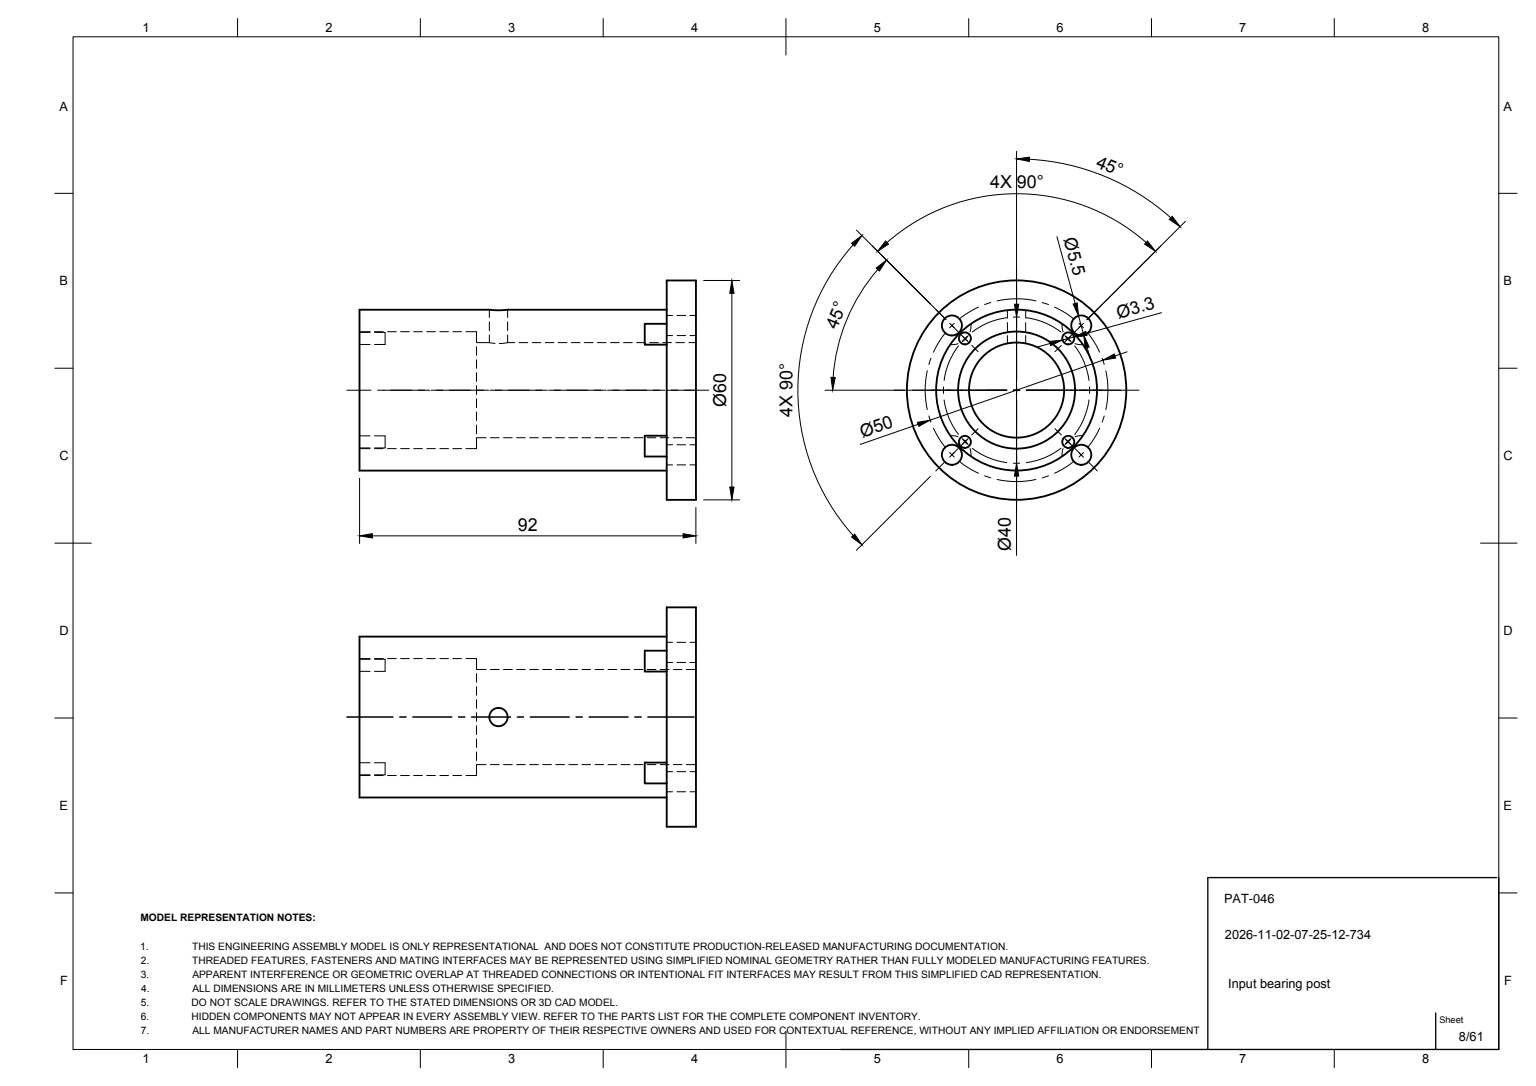
ISO-10303-21;
HEADER;
/* Generated by software containing ST-Developer
 * from STEP Tools, Inc. (www.steptools.com) 
 */

FILE_DESCRIPTION(
/* description */ ('Gear mesh backlash fixture'),
/* implementation_level */ '2;1');

FILE_NAME(
/* name */ 'Input bearing post.step',
/* time_stamp */ '2026-10-28T03:26:00-07:00',
/* author */ (''),
/* organization */ (''),
/* preprocessor_version */ 'ST-DEVELOPER v20.2',
/* originating_system */ 'Autodesk Translation Framework v15.17.0.0',
/* authorisation */ '');

FILE_SCHEMA (('AUTOMOTIVE_DESIGN { 1 0 10303 214 3 1 1 }'));
ENDSEC;

DATA;
#10=MECHANICAL_DESIGN_GEOMETRIC_PRESENTATION_REPRESENTATION('',(#1019),#57900);
#784=B_SPLINE_CURVE_WITH_KNOTS('',3,(#19392,#19393,#19394,#19395,#19396,
#19397,#19398,#19399,#19400,#19401),.UNSPECIFIED.,.F.,.F.,(4,2,2,2,4),(0.,
0.0944273339541119,0.188854667908224,0.283277491997423,0.377700316086621),
 .UNSPECIFIED.);
#785=B_SPLINE_CURVE_WITH_KNOTS('',3,(#19402,#19403,#19404,#19405,#19406,
#19407,#19408,#19409,#19410,#19411,#19412,#19413,#19414,#19415,#19416,#19417,
#19418,#19419,#19420,#19421,#19422,#19423,#19424,#19425,#19426,#19427),
 .UNSPECIFIED.,.F.,.F.,(4,2,2,2,2,2,2,2,2,2,2,2,4),(0.377700316086621,0.47212314017582,
0.56654596426502,0.660973298219131,0.755400632173242,0.849827966127354,
0.944255300081465,1.03867812417066,1.13310094825986,1.22752377234906,1.32194659643826,
1.41637393039237,1.51080126434648),.UNSPECIFIED.);
#786=B_SPLINE_CURVE_WITH_KNOTS('',3,(#19431,#19432,#19433,#19434,#19435,
#19436,#19437,#19438,#19439,#19440,#19441,#19442,#19443,#19444,#19445,#19446,
#19447,#19448,#19449,#19450,#19451,#19452,#19453,#19454,#19455,#19456),
 .UNSPECIFIED.,.F.,.F.,(4,2,2,2,2,2,2,2,2,2,2,2,4),(0.,0.0942593862034407,
0.188518772406881,0.282777622143722,0.377036471880563,0.471295321617403,
0.565554171354244,0.659813557557685,0.754072943761126,0.848332329964567,
0.942591716168009,1.03685056590485,1.13110941564169),.UNSPECIFIED.);
#787=B_SPLINE_CURVE_WITH_KNOTS('',3,(#19457,#19458,#19459,#19460,#19461,
#19462,#19463,#19464,#19465,#19466),.UNSPECIFIED.,.F.,.F.,(4,2,2,2,4),(1.13110941564169,
1.22536826537853,1.31962711511537,1.41388650131881,1.50814588752225),
 .UNSPECIFIED.);
#919=SHAPE_REPRESENTATION_RELATIONSHIP('SRR','None',#58114,#969);
#969=ADVANCED_BREP_SHAPE_REPRESENTATION('',(#1084),#57847);
#1019=STYLED_ITEM('',(#58465),#1084);
#1084=MANIFOLD_SOLID_BREP('Body1',#13579);
#1167=FACE_BOUND('',#2531,.T.);
#1168=FACE_BOUND('',#2533,.T.);
#1169=FACE_BOUND('',#2534,.T.);
#1170=FACE_BOUND('',#2535,.T.);
#1171=FACE_BOUND('',#2536,.T.);
#1172=FACE_BOUND('',#2537,.T.);
#1173=FACE_BOUND('',#2544,.T.);
#1174=FACE_BOUND('',#2547,.T.);
#1175=FACE_BOUND('',#2549,.T.);
#1176=FACE_BOUND('',#2550,.T.);
#1177=FACE_BOUND('',#2551,.T.);
#1178=FACE_BOUND('',#2552,.T.);
#1179=FACE_BOUND('',#2553,.T.);
#1180=FACE_BOUND('',#2555,.T.);
#1181=FACE_BOUND('',#2556,.T.);
#1182=FACE_BOUND('',#2557,.T.);
#1183=FACE_BOUND('',#2558,.T.);
#1184=FACE_BOUND('',#2559,.T.);
#1348=PLANE('',#14259);
#1349=PLANE('',#14263);
#1350=PLANE('',#14267);
#1351=PLANE('',#14271);
#1352=PLANE('',#14272);
#1353=PLANE('',#14280);
#1354=PLANE('',#14285);
#1355=PLANE('',#14290);
#1356=PLANE('',#14299);
#1357=PLANE('',#14316);
#1358=PLANE('',#14322);
#1359=PLANE('',#14323);
#1724=FACE_OUTER_BOUND('',#2513,.T.);
#1725=FACE_OUTER_BOUND('',#2514,.T.);
#1726=FACE_OUTER_BOUND('',#2515,.T.);
#1727=FACE_OUTER_BOUND('',#2516,.T.);
#1728=FACE_OUTER_BOUND('',#2517,.T.);
#1729=FACE_OUTER_BOUND('',#2518,.T.);
#1730=FACE_OUTER_BOUND('',#2519,.T.);
#1731=FACE_OUTER_BOUND('',#2520,.T.);
#1732=FACE_OUTER_BOUND('',#2521,.T.);
#1733=FACE_OUTER_BOUND('',#2522,.T.);
#1734=FACE_OUTER_BOUND('',#2523,.T.);
#1735=FACE_OUTER_BOUND('',#2524,.T.);
#1736=FACE_OUTER_BOUND('',#2525,.T.);
#1737=FACE_OUTER_BOUND('',#2526,.T.);
#1738=FACE_OUTER_BOUND('',#2527,.T.);
#1739=FACE_OUTER_BOUND('',#2528,.T.);
#1740=FACE_OUTER_BOUND('',#2529,.T.);
#1741=FACE_OUTER_BOUND('',#2530,.T.);
#1742=FACE_OUTER_BOUND('',#2532,.T.);
#1743=FACE_OUTER_BOUND('',#2538,.T.);
#1744=FACE_OUTER_BOUND('',#2539,.T.);
#1745=FACE_OUTER_BOUND('',#2540,.T.);
#1746=FACE_OUTER_BOUND('',#2541,.T.);
#1747=FACE_OUTER_BOUND('',#2542,.T.);
#1748=FACE_OUTER_BOUND('',#2543,.T.);
#1749=FACE_OUTER_BOUND('',#2545,.T.);
#1750=FACE_OUTER_BOUND('',#2546,.T.);
#1751=FACE_OUTER_BOUND('',#2548,.T.);
#1752=FACE_OUTER_BOUND('',#2554,.T.);
#2513=EDGE_LOOP('',(#9023,#9024,#9025,#9026,#9027,#9028));
#2514=EDGE_LOOP('',(#9029,#9030,#9031,#9032));
#2515=EDGE_LOOP('',(#9033));
#2516=EDGE_LOOP('',(#9034,#9035,#9036,#9037));
#2517=EDGE_LOOP('',(#9038));
#2518=EDGE_LOOP('',(#9039,#9040,#9041,#9042));
#2519=EDGE_LOOP('',(#9043));
#2520=EDGE_LOOP('',(#9044,#9045,#9046,#9047));
#2521=EDGE_LOOP('',(#9048));
#2522=EDGE_LOOP('',(#9049,#9050));
#2523=EDGE_LOOP('',(#9051,#9052,#9053,#9054));
#2524=EDGE_LOOP('',(#9055,#9056,#9057,#9058));
#2525=EDGE_LOOP('',(#9059,#9060));
#2526=EDGE_LOOP('',(#9061,#9062,#9063,#9064));
#2527=EDGE_LOOP('',(#9065,#9066));
#2528=EDGE_LOOP('',(#9067,#9068,#9069,#9070));
#2529=EDGE_LOOP('',(#9071,#9072));
#2530=EDGE_LOOP('',(#9073,#9074,#9075,#9076,#9077,#9078,#9079,#9080,#9081,
#9082,#9083,#9084,#9085,#9086,#9087,#9088,#9089,#9090,#9091,#9092));
#2531=EDGE_LOOP('',(#9093,#9094));
#2532=EDGE_LOOP('',(#9095));
#2533=EDGE_LOOP('',(#9096,#9097,#9098,#9099,#9100,#9101,#9102,#9103,#9104));
#2534=EDGE_LOOP('',(#9105));
#2535=EDGE_LOOP('',(#9106));
#2536=EDGE_LOOP('',(#9107));
#2537=EDGE_LOOP('',(#9108));
#2538=EDGE_LOOP('',(#9109,#9110,#9111,#9112));
#2539=EDGE_LOOP('',(#9113,#9114,#9115,#9116));
#2540=EDGE_LOOP('',(#9117,#9118,#9119,#9120));
#2541=EDGE_LOOP('',(#9121,#9122,#9123,#9124));
#2542=EDGE_LOOP('',(#9125,#9126,#9127,#9128));
#2543=EDGE_LOOP('',(#9129));
#2544=EDGE_LOOP('',(#9130));
#2545=EDGE_LOOP('',(#9131,#9132,#9133,#9134));
#2546=EDGE_LOOP('',(#9135,#9136,#9137,#9138));
#2547=EDGE_LOOP('',(#9139,#9140));
#2548=EDGE_LOOP('',(#9141));
#2549=EDGE_LOOP('',(#9142));
#2550=EDGE_LOOP('',(#9143));
#2551=EDGE_LOOP('',(#9144));
#2552=EDGE_LOOP('',(#9145));
#2553=EDGE_LOOP('',(#9146));
#2554=EDGE_LOOP('',(#9147));
#2555=EDGE_LOOP('',(#9148));
#2556=EDGE_LOOP('',(#9149));
#2557=EDGE_LOOP('',(#9150));
#2558=EDGE_LOOP('',(#9151));
#2559=EDGE_LOOP('',(#9152));
#3459=LINE('',#19429,#4348);
#3460=LINE('',#19471,#4349);
#3461=LINE('',#19478,#4350);
#3462=LINE('',#19485,#4351);
#3463=LINE('',#19492,#4352);
#3464=LINE('',#19502,#4353);
#3465=LINE('',#19505,#4354);
#3466=LINE('',#19509,#4355);
#3467=LINE('',#19513,#4356);
#3468=LINE('',#19520,#4357);
#3469=LINE('',#19524,#4358);
#3470=LINE('',#19531,#4359);
#3471=LINE('',#19535,#4360);
#3472=LINE('',#19543,#4361);
#3473=LINE('',#19563,#4362);
#3474=LINE('',#19567,#4363);
#3475=LINE('',#19571,#4364);
#3476=LINE('',#19575,#4365);
#3477=LINE('',#19580,#4366);
#3478=LINE('',#19587,#4367);
#3479=LINE('',#19591,#4368);
#4348=VECTOR('',#15748,0.25);
#4349=VECTOR('',#15753,0.165);
#4350=VECTOR('',#15762,0.165);
#4351=VECTOR('',#15771,0.165);
#4352=VECTOR('',#15780,0.165);
#4353=VECTOR('',#15793,1.);
#4354=VECTOR('',#15796,1.);
#4355=VECTOR('',#15799,1.);
#4356=VECTOR('',#15802,1.);
#4357=VECTOR('',#15811,1.);
#4358=VECTOR('',#15814,1.);
#4359=VECTOR('',#15823,1.);
#4360=VECTOR('',#15826,1.);
#4361=VECTOR('',#15837,2.2);
#4362=VECTOR('',#15864,0.275);
#4363=VECTOR('',#15869,0.275);
#4364=VECTOR('',#15874,0.275);
#4365=VECTOR('',#15879,0.275);
#4366=VECTOR('',#15884,1.6);
#4367=VECTOR('',#15893,3.);
#4368=VECTOR('',#15898,1.3);
#5213=CIRCLE('',#14257,0.165);
#5214=CIRCLE('',#14258,0.165);
#5215=CIRCLE('',#14261,0.165);
#5216=CIRCLE('',#14262,0.165);
#5217=CIRCLE('',#14265,0.165);
#5218=CIRCLE('',#14266,0.165);
#5219=CIRCLE('',#14269,0.165);
#5220=CIRCLE('',#14270,0.165);
#5221=CIRCLE('',#14273,2.2);
#5222=CIRCLE('',#14274,0.525);
#5223=CIRCLE('',#14276,0.525);
#5224=CIRCLE('',#14278,0.525);
#5225=CIRCLE('',#14279,0.525);
#5226=CIRCLE('',#14281,2.2);
#5227=CIRCLE('',#14283,0.525);
#5228=CIRCLE('',#14284,0.525);
#5229=CIRCLE('',#14286,2.2);
#5230=CIRCLE('',#14288,0.525);
#5231=CIRCLE('',#14289,0.525);
#5232=CIRCLE('',#14291,2.2);
#5233=CIRCLE('',#14293,2.2);
#5234=CIRCLE('',#14294,2.2);
#5235=CIRCLE('',#14295,2.2);
#5236=CIRCLE('',#14296,2.2);
#5237=CIRCLE('',#14297,2.2);
#5238=CIRCLE('',#14298,2.2);
#5239=CIRCLE('',#14300,3.);
#5240=CIRCLE('',#14301,0.275);
#5241=CIRCLE('',#14302,0.275);
#5242=CIRCLE('',#14303,0.275);
#5243=CIRCLE('',#14304,0.275);
#5244=CIRCLE('',#14306,0.275);
#5245=CIRCLE('',#14308,0.275);
#5246=CIRCLE('',#14310,0.275);
#5247=CIRCLE('',#14312,0.275);
#5248=CIRCLE('',#14314,1.6);
#5249=CIRCLE('',#14315,1.6);
#5250=CIRCLE('',#14317,1.3);
#5251=CIRCLE('',#14319,3.);
#5252=CIRCLE('',#14321,1.3);
#5829=VERTEX_POINT('',#19390);
#5830=VERTEX_POINT('',#19391);
#5831=VERTEX_POINT('',#19428);
#5832=VERTEX_POINT('',#19430);
#5833=VERTEX_POINT('',#19468);
#5834=VERTEX_POINT('',#19470);
#5835=VERTEX_POINT('',#19475);
#5836=VERTEX_POINT('',#19477);
#5837=VERTEX_POINT('',#19482);
#5838=VERTEX_POINT('',#19484);
#5839=VERTEX_POINT('',#19489);
#5840=VERTEX_POINT('',#19491);
#5841=VERTEX_POINT('',#19496);
#5842=VERTEX_POINT('',#19497);
#5843=VERTEX_POINT('',#19501);
#5844=VERTEX_POINT('',#19503);
#5845=VERTEX_POINT('',#19507);
#5846=VERTEX_POINT('',#19508);
#5847=VERTEX_POINT('',#19510);
#5848=VERTEX_POINT('',#19512);
#5849=VERTEX_POINT('',#19518);
#5850=VERTEX_POINT('',#19519);
#5851=VERTEX_POINT('',#19521);
#5852=VERTEX_POINT('',#19523);
#5853=VERTEX_POINT('',#19529);
#5854=VERTEX_POINT('',#19530);
#5855=VERTEX_POINT('',#19532);
#5856=VERTEX_POINT('',#19534);
#5857=VERTEX_POINT('',#19540);
#5858=VERTEX_POINT('',#19542);
#5859=VERTEX_POINT('',#19550);
#5860=VERTEX_POINT('',#19552);
#5861=VERTEX_POINT('',#19554);
#5862=VERTEX_POINT('',#19556);
#5863=VERTEX_POINT('',#19558);
#5864=VERTEX_POINT('',#19561);
#5865=VERTEX_POINT('',#19565);
#5866=VERTEX_POINT('',#19569);
#5867=VERTEX_POINT('',#19573);
#5868=VERTEX_POINT('',#19577);
#5869=VERTEX_POINT('',#19579);
#5870=VERTEX_POINT('',#19583);
#5871=VERTEX_POINT('',#19586);
#5872=VERTEX_POINT('',#19590);
#7098=EDGE_CURVE('',#5829,#5830,#784,.T.);
#7099=EDGE_CURVE('',#5830,#5829,#785,.T.);
#7100=EDGE_CURVE('',#5830,#5831,#3459,.T.);
#7101=EDGE_CURVE('',#5832,#5831,#786,.T.);
#7102=EDGE_CURVE('',#5831,#5832,#787,.T.);
#7103=EDGE_CURVE('',#5833,#5833,#5213,.T.);
#7104=EDGE_CURVE('',#5833,#5834,#3460,.T.);
#7105=EDGE_CURVE('',#5834,#5834,#5214,.T.);
#7106=EDGE_CURVE('',#5835,#5835,#5215,.T.);
#7107=EDGE_CURVE('',#5835,#5836,#3461,.T.);
#7108=EDGE_CURVE('',#5836,#5836,#5216,.T.);
#7109=EDGE_CURVE('',#5837,#5837,#5217,.T.);
#7110=EDGE_CURVE('',#5837,#5838,#3462,.T.);
#7111=EDGE_CURVE('',#5838,#5838,#5218,.T.);
#7112=EDGE_CURVE('',#5839,#5839,#5219,.T.);
#7113=EDGE_CURVE('',#5839,#5840,#3463,.T.);
#7114=EDGE_CURVE('',#5840,#5840,#5220,.T.);
#7115=EDGE_CURVE('',#5841,#5842,#5221,.T.);
#7116=EDGE_CURVE('',#5842,#5841,#5222,.T.);
#7117=EDGE_CURVE('',#5843,#5841,#3464,.T.);
#7118=EDGE_CURVE('',#5844,#5843,#5223,.T.);
#7119=EDGE_CURVE('',#5842,#5844,#3465,.T.);
#7120=EDGE_CURVE('',#5845,#5846,#3466,.T.);
#7121=EDGE_CURVE('',#5845,#5847,#5224,.T.);
#7122=EDGE_CURVE('',#5848,#5847,#3467,.T.);
#7123=EDGE_CURVE('',#5846,#5848,#5225,.T.);
#7124=EDGE_CURVE('',#5847,#5845,#5226,.T.);
#7125=EDGE_CURVE('',#5849,#5850,#3468,.T.);
#7126=EDGE_CURVE('',#5849,#5851,#5227,.T.);
#7127=EDGE_CURVE('',#5852,#5851,#3469,.T.);
#7128=EDGE_CURVE('',#5850,#5852,#5228,.T.);
#7129=EDGE_CURVE('',#5851,#5849,#5229,.T.);
#7130=EDGE_CURVE('',#5853,#5854,#3470,.T.);
#7131=EDGE_CURVE('',#5853,#5855,#5230,.T.);
#7132=EDGE_CURVE('',#5856,#5855,#3471,.T.);
#7133=EDGE_CURVE('',#5854,#5856,#5231,.T.);
#7134=EDGE_CURVE('',#5855,#5853,#5232,.T.);
#7135=EDGE_CURVE('',#5857,#5857,#5233,.T.);
#7136=EDGE_CURVE('',#5857,#5858,#3472,.T.);
#7137=EDGE_CURVE('',#5858,#5843,#5234,.T.);
#7138=EDGE_CURVE('',#5844,#5856,#5235,.T.);
#7139=EDGE_CURVE('',#5854,#5852,#5236,.T.);
#7140=EDGE_CURVE('',#5850,#5848,#5237,.T.);
#7141=EDGE_CURVE('',#5846,#5858,#5238,.T.);
#7142=EDGE_CURVE('',#5859,#5859,#5239,.T.);
#7143=EDGE_CURVE('',#5860,#5860,#5240,.T.);
#7144=EDGE_CURVE('',#5861,#5861,#5241,.T.);
#7145=EDGE_CURVE('',#5862,#5862,#5242,.T.);
#7146=EDGE_CURVE('',#5863,#5863,#5243,.T.);
#7147=EDGE_CURVE('',#5864,#5864,#5244,.T.);
#7148=EDGE_CURVE('',#5864,#5860,#3473,.T.);
#7149=EDGE_CURVE('',#5865,#5865,#5245,.T.);
#7150=EDGE_CURVE('',#5865,#5863,#3474,.T.);
#7151=EDGE_CURVE('',#5866,#5866,#5246,.T.);
#7152=EDGE_CURVE('',#5866,#5861,#3475,.T.);
#7153=EDGE_CURVE('',#5867,#5867,#5247,.T.);
#7154=EDGE_CURVE('',#5867,#5862,#3476,.T.);
#7155=EDGE_CURVE('',#5868,#5868,#5248,.T.);
#7156=EDGE_CURVE('',#5868,#5869,#3477,.T.);
#7157=EDGE_CURVE('',#5869,#5869,#5249,.T.);
#7158=EDGE_CURVE('',#5870,#5870,#5250,.T.);
#7159=EDGE_CURVE('',#5859,#5871,#3478,.T.);
#7160=EDGE_CURVE('',#5871,#5871,#5251,.T.);
#7161=EDGE_CURVE('',#5870,#5872,#3479,.T.);
#7162=EDGE_CURVE('',#5872,#5872,#5252,.T.);
#9023=ORIENTED_EDGE('',*,*,#7098,.F.);
#9024=ORIENTED_EDGE('',*,*,#7099,.F.);
#9025=ORIENTED_EDGE('',*,*,#7100,.T.);
#9026=ORIENTED_EDGE('',*,*,#7101,.F.);
#9027=ORIENTED_EDGE('',*,*,#7102,.F.);
#9028=ORIENTED_EDGE('',*,*,#7100,.F.);
#9029=ORIENTED_EDGE('',*,*,#7103,.F.);
#9030=ORIENTED_EDGE('',*,*,#7104,.T.);
#9031=ORIENTED_EDGE('',*,*,#7105,.F.);
#9032=ORIENTED_EDGE('',*,*,#7104,.F.);
#9033=ORIENTED_EDGE('',*,*,#7103,.T.);
#9034=ORIENTED_EDGE('',*,*,#7106,.F.);
#9035=ORIENTED_EDGE('',*,*,#7107,.T.);
#9036=ORIENTED_EDGE('',*,*,#7108,.F.);
#9037=ORIENTED_EDGE('',*,*,#7107,.F.);
#9038=ORIENTED_EDGE('',*,*,#7106,.T.);
#9039=ORIENTED_EDGE('',*,*,#7109,.F.);
#9040=ORIENTED_EDGE('',*,*,#7110,.T.);
#9041=ORIENTED_EDGE('',*,*,#7111,.F.);
#9042=ORIENTED_EDGE('',*,*,#7110,.F.);
#9043=ORIENTED_EDGE('',*,*,#7109,.T.);
#9044=ORIENTED_EDGE('',*,*,#7112,.F.);
#9045=ORIENTED_EDGE('',*,*,#7113,.T.);
#9046=ORIENTED_EDGE('',*,*,#7114,.F.);
#9047=ORIENTED_EDGE('',*,*,#7113,.F.);
#9048=ORIENTED_EDGE('',*,*,#7112,.T.);
#9049=ORIENTED_EDGE('',*,*,#7115,.F.);
#9050=ORIENTED_EDGE('',*,*,#7116,.F.);
#9051=ORIENTED_EDGE('',*,*,#7117,.F.);
#9052=ORIENTED_EDGE('',*,*,#7118,.F.);
#9053=ORIENTED_EDGE('',*,*,#7119,.F.);
#9054=ORIENTED_EDGE('',*,*,#7116,.T.);
#9055=ORIENTED_EDGE('',*,*,#7120,.F.);
#9056=ORIENTED_EDGE('',*,*,#7121,.T.);
#9057=ORIENTED_EDGE('',*,*,#7122,.F.);
#9058=ORIENTED_EDGE('',*,*,#7123,.F.);
#9059=ORIENTED_EDGE('',*,*,#7124,.F.);
#9060=ORIENTED_EDGE('',*,*,#7121,.F.);
#9061=ORIENTED_EDGE('',*,*,#7125,.F.);
#9062=ORIENTED_EDGE('',*,*,#7126,.T.);
#9063=ORIENTED_EDGE('',*,*,#7127,.F.);
#9064=ORIENTED_EDGE('',*,*,#7128,.F.);
#9065=ORIENTED_EDGE('',*,*,#7129,.F.);
#9066=ORIENTED_EDGE('',*,*,#7126,.F.);
#9067=ORIENTED_EDGE('',*,*,#7130,.F.);
#9068=ORIENTED_EDGE('',*,*,#7131,.T.);
#9069=ORIENTED_EDGE('',*,*,#7132,.F.);
#9070=ORIENTED_EDGE('',*,*,#7133,.F.);
#9071=ORIENTED_EDGE('',*,*,#7134,.F.);
#9072=ORIENTED_EDGE('',*,*,#7131,.F.);
#9073=ORIENTED_EDGE('',*,*,#7135,.F.);
#9074=ORIENTED_EDGE('',*,*,#7136,.T.);
#9075=ORIENTED_EDGE('',*,*,#7137,.T.);
#9076=ORIENTED_EDGE('',*,*,#7117,.T.);
#9077=ORIENTED_EDGE('',*,*,#7115,.T.);
#9078=ORIENTED_EDGE('',*,*,#7119,.T.);
#9079=ORIENTED_EDGE('',*,*,#7138,.T.);
#9080=ORIENTED_EDGE('',*,*,#7132,.T.);
#9081=ORIENTED_EDGE('',*,*,#7134,.T.);
#9082=ORIENTED_EDGE('',*,*,#7130,.T.);
#9083=ORIENTED_EDGE('',*,*,#7139,.T.);
#9084=ORIENTED_EDGE('',*,*,#7127,.T.);
#9085=ORIENTED_EDGE('',*,*,#7129,.T.);
#9086=ORIENTED_EDGE('',*,*,#7125,.T.);
#9087=ORIENTED_EDGE('',*,*,#7140,.T.);
#9088=ORIENTED_EDGE('',*,*,#7122,.T.);
#9089=ORIENTED_EDGE('',*,*,#7124,.T.);
#9090=ORIENTED_EDGE('',*,*,#7120,.T.);
#9091=ORIENTED_EDGE('',*,*,#7141,.T.);
#9092=ORIENTED_EDGE('',*,*,#7136,.F.);
#9093=ORIENTED_EDGE('',*,*,#7101,.T.);
#9094=ORIENTED_EDGE('',*,*,#7102,.T.);
#9095=ORIENTED_EDGE('',*,*,#7142,.T.);
#9096=ORIENTED_EDGE('',*,*,#7141,.F.);
#9097=ORIENTED_EDGE('',*,*,#7123,.T.);
#9098=ORIENTED_EDGE('',*,*,#7140,.F.);
#9099=ORIENTED_EDGE('',*,*,#7128,.T.);
#9100=ORIENTED_EDGE('',*,*,#7139,.F.);
#9101=ORIENTED_EDGE('',*,*,#7133,.T.);
#9102=ORIENTED_EDGE('',*,*,#7138,.F.);
#9103=ORIENTED_EDGE('',*,*,#7118,.T.);
#9104=ORIENTED_EDGE('',*,*,#7137,.F.);
#9105=ORIENTED_EDGE('',*,*,#7143,.T.);
#9106=ORIENTED_EDGE('',*,*,#7144,.T.);
#9107=ORIENTED_EDGE('',*,*,#7145,.T.);
#9108=ORIENTED_EDGE('',*,*,#7146,.T.);
#9109=ORIENTED_EDGE('',*,*,#7147,.F.);
#9110=ORIENTED_EDGE('',*,*,#7148,.T.);
#9111=ORIENTED_EDGE('',*,*,#7143,.F.);
#9112=ORIENTED_EDGE('',*,*,#7148,.F.);
#9113=ORIENTED_EDGE('',*,*,#7149,.F.);
#9114=ORIENTED_EDGE('',*,*,#7150,.T.);
#9115=ORIENTED_EDGE('',*,*,#7146,.F.);
#9116=ORIENTED_EDGE('',*,*,#7150,.F.);
#9117=ORIENTED_EDGE('',*,*,#7151,.F.);
#9118=ORIENTED_EDGE('',*,*,#7152,.T.);
#9119=ORIENTED_EDGE('',*,*,#7144,.F.);
#9120=ORIENTED_EDGE('',*,*,#7152,.F.);
#9121=ORIENTED_EDGE('',*,*,#7153,.F.);
#9122=ORIENTED_EDGE('',*,*,#7154,.T.);
#9123=ORIENTED_EDGE('',*,*,#7145,.F.);
#9124=ORIENTED_EDGE('',*,*,#7154,.F.);
#9125=ORIENTED_EDGE('',*,*,#7155,.F.);
#9126=ORIENTED_EDGE('',*,*,#7156,.T.);
#9127=ORIENTED_EDGE('',*,*,#7157,.F.);
#9128=ORIENTED_EDGE('',*,*,#7156,.F.);
#9129=ORIENTED_EDGE('',*,*,#7155,.T.);
#9130=ORIENTED_EDGE('',*,*,#7158,.F.);
#9131=ORIENTED_EDGE('',*,*,#7142,.F.);
#9132=ORIENTED_EDGE('',*,*,#7159,.T.);
#9133=ORIENTED_EDGE('',*,*,#7160,.T.);
#9134=ORIENTED_EDGE('',*,*,#7159,.F.);
#9135=ORIENTED_EDGE('',*,*,#7158,.T.);
#9136=ORIENTED_EDGE('',*,*,#7161,.T.);
#9137=ORIENTED_EDGE('',*,*,#7162,.T.);
#9138=ORIENTED_EDGE('',*,*,#7161,.F.);
#9139=ORIENTED_EDGE('',*,*,#7098,.T.);
#9140=ORIENTED_EDGE('',*,*,#7099,.T.);
#9141=ORIENTED_EDGE('',*,*,#7135,.T.);
#9142=ORIENTED_EDGE('',*,*,#7157,.T.);
#9143=ORIENTED_EDGE('',*,*,#7114,.T.);
#9144=ORIENTED_EDGE('',*,*,#7111,.T.);
#9145=ORIENTED_EDGE('',*,*,#7108,.T.);
#9146=ORIENTED_EDGE('',*,*,#7105,.T.);
#9147=ORIENTED_EDGE('',*,*,#7160,.F.);
#9148=ORIENTED_EDGE('',*,*,#7162,.F.);
#9149=ORIENTED_EDGE('',*,*,#7153,.T.);
#9150=ORIENTED_EDGE('',*,*,#7151,.T.);
#9151=ORIENTED_EDGE('',*,*,#7149,.T.);
#9152=ORIENTED_EDGE('',*,*,#7147,.T.);
#12597=CYLINDRICAL_SURFACE('',#14255,0.25);
#12598=CYLINDRICAL_SURFACE('',#14256,0.165);
#12599=CYLINDRICAL_SURFACE('',#14260,0.165);
#12600=CYLINDRICAL_SURFACE('',#14264,0.165);
#12601=CYLINDRICAL_SURFACE('',#14268,0.165);
#12602=CYLINDRICAL_SURFACE('',#14275,0.525);
#12603=CYLINDRICAL_SURFACE('',#14277,0.525);
#12604=CYLINDRICAL_SURFACE('',#14282,0.525);
#12605=CYLINDRICAL_SURFACE('',#14287,0.525);
#12606=CYLINDRICAL_SURFACE('',#14292,2.2);
#12607=CYLINDRICAL_SURFACE('',#14305,0.275);
#12608=CYLINDRICAL_SURFACE('',#14307,0.275);
#12609=CYLINDRICAL_SURFACE('',#14309,0.275);
#12610=CYLINDRICAL_SURFACE('',#14311,0.275);
#12611=CYLINDRICAL_SURFACE('',#14313,1.6);
#12612=CYLINDRICAL_SURFACE('',#14318,3.);
#12613=CYLINDRICAL_SURFACE('',#14320,1.3);
#12841=ADVANCED_FACE('',(#1724),#12597,.F.);
#12842=ADVANCED_FACE('',(#1725),#12598,.F.);
#12843=ADVANCED_FACE('',(#1726),#1348,.T.);
#12844=ADVANCED_FACE('',(#1727),#12599,.F.);
#12845=ADVANCED_FACE('',(#1728),#1349,.T.);
#12846=ADVANCED_FACE('',(#1729),#12600,.F.);
#12847=ADVANCED_FACE('',(#1730),#1350,.T.);
#12848=ADVANCED_FACE('',(#1731),#12601,.F.);
#12849=ADVANCED_FACE('',(#1732),#1351,.T.);
#12850=ADVANCED_FACE('',(#1733),#1352,.F.);
#12851=ADVANCED_FACE('',(#1734),#12602,.F.);
#12852=ADVANCED_FACE('',(#1735),#12603,.F.);
#12853=ADVANCED_FACE('',(#1736),#1353,.F.);
#12854=ADVANCED_FACE('',(#1737),#12604,.F.);
#12855=ADVANCED_FACE('',(#1738),#1354,.F.);
#12856=ADVANCED_FACE('',(#1739),#12605,.F.);
#12857=ADVANCED_FACE('',(#1740),#1355,.F.);
#12858=ADVANCED_FACE('',(#1741,#1167),#12606,.T.);
#12859=ADVANCED_FACE('',(#1742,#1168,#1169,#1170,#1171,#1172),#1356,.T.);
#12860=ADVANCED_FACE('',(#1743),#12607,.F.);
#12861=ADVANCED_FACE('',(#1744),#12608,.F.);
#12862=ADVANCED_FACE('',(#1745),#12609,.F.);
#12863=ADVANCED_FACE('',(#1746),#12610,.F.);
#12864=ADVANCED_FACE('',(#1747),#12611,.F.);
#12865=ADVANCED_FACE('',(#1748,#1173),#1357,.T.);
#12866=ADVANCED_FACE('',(#1749),#12612,.T.);
#12867=ADVANCED_FACE('',(#1750,#1174),#12613,.F.);
#12868=ADVANCED_FACE('',(#1751,#1175,#1176,#1177,#1178,#1179),#1358,.T.);
#12869=ADVANCED_FACE('',(#1752,#1180,#1181,#1182,#1183,#1184),#1359,.F.);
#13579=CLOSED_SHELL('',(#12841,#12842,#12843,#12844,#12845,#12846,#12847,
#12848,#12849,#12850,#12851,#12852,#12853,#12854,#12855,#12856,#12857,#12858,
#12859,#12860,#12861,#12862,#12863,#12864,#12865,#12866,#12867,#12868,#12869));
#14254=AXIS2_PLACEMENT_3D('',#19388,#15744,#15745);
#14255=AXIS2_PLACEMENT_3D('',#19389,#15746,#15747);
#14256=AXIS2_PLACEMENT_3D('',#19467,#15749,#15750);
#14257=AXIS2_PLACEMENT_3D('',#19469,#15751,#15752);
#14258=AXIS2_PLACEMENT_3D('',#19472,#15754,#15755);
#14259=AXIS2_PLACEMENT_3D('',#19473,#15756,#15757);
#14260=AXIS2_PLACEMENT_3D('',#19474,#15758,#15759);
#14261=AXIS2_PLACEMENT_3D('',#19476,#15760,#15761);
#14262=AXIS2_PLACEMENT_3D('',#19479,#15763,#15764);
#14263=AXIS2_PLACEMENT_3D('',#19480,#15765,#15766);
#14264=AXIS2_PLACEMENT_3D('',#19481,#15767,#15768);
#14265=AXIS2_PLACEMENT_3D('',#19483,#15769,#15770);
#14266=AXIS2_PLACEMENT_3D('',#19486,#15772,#15773);
#14267=AXIS2_PLACEMENT_3D('',#19487,#15774,#15775);
#14268=AXIS2_PLACEMENT_3D('',#19488,#15776,#15777);
#14269=AXIS2_PLACEMENT_3D('',#19490,#15778,#15779);
#14270=AXIS2_PLACEMENT_3D('',#19493,#15781,#15782);
#14271=AXIS2_PLACEMENT_3D('',#19494,#15783,#15784);
#14272=AXIS2_PLACEMENT_3D('',#19495,#15785,#15786);
#14273=AXIS2_PLACEMENT_3D('',#19498,#15787,#15788);
#14274=AXIS2_PLACEMENT_3D('',#19499,#15789,#15790);
#14275=AXIS2_PLACEMENT_3D('',#19500,#15791,#15792);
#14276=AXIS2_PLACEMENT_3D('',#19504,#15794,#15795);
#14277=AXIS2_PLACEMENT_3D('',#19506,#15797,#15798);
#14278=AXIS2_PLACEMENT_3D('',#19511,#15800,#15801);
#14279=AXIS2_PLACEMENT_3D('',#19514,#15803,#15804);
#14280=AXIS2_PLACEMENT_3D('',#19515,#15805,#15806);
#14281=AXIS2_PLACEMENT_3D('',#19516,#15807,#15808);
#14282=AXIS2_PLACEMENT_3D('',#19517,#15809,#15810);
#14283=AXIS2_PLACEMENT_3D('',#19522,#15812,#15813);
#14284=AXIS2_PLACEMENT_3D('',#19525,#15815,#15816);
#14285=AXIS2_PLACEMENT_3D('',#19526,#15817,#15818);
#14286=AXIS2_PLACEMENT_3D('',#19527,#15819,#15820);
#14287=AXIS2_PLACEMENT_3D('',#19528,#15821,#15822);
#14288=AXIS2_PLACEMENT_3D('',#19533,#15824,#15825);
#14289=AXIS2_PLACEMENT_3D('',#19536,#15827,#15828);
#14290=AXIS2_PLACEMENT_3D('',#19537,#15829,#15830);
#14291=AXIS2_PLACEMENT_3D('',#19538,#15831,#15832);
#14292=AXIS2_PLACEMENT_3D('',#19539,#15833,#15834);
#14293=AXIS2_PLACEMENT_3D('',#19541,#15835,#15836);
#14294=AXIS2_PLACEMENT_3D('',#19544,#15838,#15839);
#14295=AXIS2_PLACEMENT_3D('',#19545,#15840,#15841);
#14296=AXIS2_PLACEMENT_3D('',#19546,#15842,#15843);
#14297=AXIS2_PLACEMENT_3D('',#19547,#15844,#15845);
#14298=AXIS2_PLACEMENT_3D('',#19548,#15846,#15847);
#14299=AXIS2_PLACEMENT_3D('',#19549,#15848,#15849);
#14300=AXIS2_PLACEMENT_3D('',#19551,#15850,#15851);
#14301=AXIS2_PLACEMENT_3D('',#19553,#15852,#15853);
#14302=AXIS2_PLACEMENT_3D('',#19555,#15854,#15855);
#14303=AXIS2_PLACEMENT_3D('',#19557,#15856,#15857);
#14304=AXIS2_PLACEMENT_3D('',#19559,#15858,#15859);
#14305=AXIS2_PLACEMENT_3D('',#19560,#15860,#15861);
#14306=AXIS2_PLACEMENT_3D('',#19562,#15862,#15863);
#14307=AXIS2_PLACEMENT_3D('',#19564,#15865,#15866);
#14308=AXIS2_PLACEMENT_3D('',#19566,#15867,#15868);
#14309=AXIS2_PLACEMENT_3D('',#19568,#15870,#15871);
#14310=AXIS2_PLACEMENT_3D('',#19570,#15872,#15873);
#14311=AXIS2_PLACEMENT_3D('',#19572,#15875,#15876);
#14312=AXIS2_PLACEMENT_3D('',#19574,#15877,#15878);
#14313=AXIS2_PLACEMENT_3D('',#19576,#15880,#15881);
#14314=AXIS2_PLACEMENT_3D('',#19578,#15882,#15883);
#14315=AXIS2_PLACEMENT_3D('',#19581,#15885,#15886);
#14316=AXIS2_PLACEMENT_3D('',#19582,#15887,#15888);
#14317=AXIS2_PLACEMENT_3D('',#19584,#15889,#15890);
#14318=AXIS2_PLACEMENT_3D('',#19585,#15891,#15892);
#14319=AXIS2_PLACEMENT_3D('',#19588,#15894,#15895);
#14320=AXIS2_PLACEMENT_3D('',#19589,#15896,#15897);
#14321=AXIS2_PLACEMENT_3D('',#19592,#15899,#15900);
#14322=AXIS2_PLACEMENT_3D('',#19593,#15901,#15902);
#14323=AXIS2_PLACEMENT_3D('',#19594,#15903,#15904);
#15744=DIRECTION('axis',(0.,0.,1.));
#15745=DIRECTION('refdir',(1.,0.,0.));
#15746=DIRECTION('center_axis',(1.,0.,0.));
#15747=DIRECTION('ref_axis',(0.,0.,-1.));
#15748=DIRECTION('',(1.,0.,0.));
#15749=DIRECTION('center_axis',(0.,0.,1.));
#15750=DIRECTION('ref_axis',(1.,0.,0.));
#15751=DIRECTION('center_axis',(0.,0.,1.));
#15752=DIRECTION('ref_axis',(1.,0.,0.));
#15753=DIRECTION('',(0.,0.,1.));
#15754=DIRECTION('center_axis',(0.,0.,-1.));
#15755=DIRECTION('ref_axis',(1.,0.,0.));
#15756=DIRECTION('center_axis',(0.,0.,1.));
#15757=DIRECTION('ref_axis',(1.,0.,0.));
#15758=DIRECTION('center_axis',(0.,0.,1.));
#15759=DIRECTION('ref_axis',(1.,0.,0.));
#15760=DIRECTION('center_axis',(0.,0.,1.));
#15761=DIRECTION('ref_axis',(1.,0.,0.));
#15762=DIRECTION('',(0.,0.,1.));
#15763=DIRECTION('center_axis',(0.,0.,-1.));
#15764=DIRECTION('ref_axis',(1.,0.,0.));
#15765=DIRECTION('center_axis',(0.,0.,1.));
#15766=DIRECTION('ref_axis',(1.,0.,0.));
#15767=DIRECTION('center_axis',(0.,0.,1.));
#15768=DIRECTION('ref_axis',(1.,0.,0.));
#15769=DIRECTION('center_axis',(0.,0.,1.));
#15770=DIRECTION('ref_axis',(1.,0.,0.));
#15771=DIRECTION('',(0.,0.,1.));
#15772=DIRECTION('center_axis',(0.,0.,-1.));
#15773=DIRECTION('ref_axis',(1.,0.,0.));
#15774=DIRECTION('center_axis',(0.,0.,1.));
#15775=DIRECTION('ref_axis',(1.,0.,0.));
#15776=DIRECTION('center_axis',(0.,0.,1.));
#15777=DIRECTION('ref_axis',(1.,0.,0.));
#15778=DIRECTION('center_axis',(0.,0.,1.));
#15779=DIRECTION('ref_axis',(1.,0.,0.));
#15780=DIRECTION('',(0.,0.,1.));
#15781=DIRECTION('center_axis',(0.,0.,-1.));
#15782=DIRECTION('ref_axis',(1.,0.,0.));
#15783=DIRECTION('center_axis',(0.,0.,1.));
#15784=DIRECTION('ref_axis',(1.,0.,0.));
#15785=DIRECTION('center_axis',(0.,0.,1.));
#15786=DIRECTION('ref_axis',(1.,0.,0.));
#15787=DIRECTION('center_axis',(0.,0.,1.));
#15788=DIRECTION('ref_axis',(1.,0.,0.));
#15789=DIRECTION('center_axis',(0.,0.,1.));
#15790=DIRECTION('ref_axis',(1.,0.,0.));
#15791=DIRECTION('center_axis',(0.,0.,1.));
#15792=DIRECTION('ref_axis',(1.,0.,0.));
#15793=DIRECTION('',(0.,0.,1.));
#15794=DIRECTION('center_axis',(0.,0.,1.));
#15795=DIRECTION('ref_axis',(1.,0.,0.));
#15796=DIRECTION('',(0.,0.,-1.));
#15797=DIRECTION('center_axis',(0.,0.,1.));
#15798=DIRECTION('ref_axis',(1.,0.,0.));
#15799=DIRECTION('',(0.,0.,-1.));
#15800=DIRECTION('center_axis',(0.,0.,1.));
#15801=DIRECTION('ref_axis',(1.,0.,0.));
#15802=DIRECTION('',(0.,0.,1.));
#15803=DIRECTION('center_axis',(0.,0.,1.));
#15804=DIRECTION('ref_axis',(1.,0.,0.));
#15805=DIRECTION('center_axis',(0.,0.,1.));
#15806=DIRECTION('ref_axis',(1.,0.,0.));
#15807=DIRECTION('center_axis',(0.,0.,1.));
#15808=DIRECTION('ref_axis',(1.,0.,0.));
#15809=DIRECTION('center_axis',(0.,0.,1.));
#15810=DIRECTION('ref_axis',(-0.707106781186548,-0.707106781186547,0.));
#15811=DIRECTION('',(0.,0.,-1.));
#15812=DIRECTION('center_axis',(0.,0.,1.));
#15813=DIRECTION('ref_axis',(1.,0.,0.));
#15814=DIRECTION('',(0.,0.,1.));
#15815=DIRECTION('center_axis',(0.,0.,1.));
#15816=DIRECTION('ref_axis',(1.,0.,0.));
#15817=DIRECTION('center_axis',(0.,0.,1.));
#15818=DIRECTION('ref_axis',(1.,0.,0.));
#15819=DIRECTION('center_axis',(0.,0.,1.));
#15820=DIRECTION('ref_axis',(1.,0.,0.));
#15821=DIRECTION('center_axis',(0.,0.,1.));
#15822=DIRECTION('ref_axis',(-0.707106781186547,0.707106781186548,0.));
#15823=DIRECTION('',(0.,0.,-1.));
#15824=DIRECTION('center_axis',(0.,0.,1.));
#15825=DIRECTION('ref_axis',(1.,0.,0.));
#15826=DIRECTION('',(0.,0.,1.));
#15827=DIRECTION('center_axis',(0.,0.,1.));
#15828=DIRECTION('ref_axis',(1.,0.,0.));
#15829=DIRECTION('center_axis',(0.,0.,1.));
#15830=DIRECTION('ref_axis',(1.,0.,0.));
#15831=DIRECTION('center_axis',(0.,0.,1.));
#15832=DIRECTION('ref_axis',(1.,0.,0.));
#15833=DIRECTION('center_axis',(0.,0.,1.));
#15834=DIRECTION('ref_axis',(1.,0.,0.));
#15835=DIRECTION('center_axis',(0.,0.,1.));
#15836=DIRECTION('ref_axis',(1.,0.,0.));
#15837=DIRECTION('',(0.,0.,-1.));
#15838=DIRECTION('center_axis',(0.,0.,1.));
#15839=DIRECTION('ref_axis',(1.,0.,0.));
#15840=DIRECTION('center_axis',(0.,0.,1.));
#15841=DIRECTION('ref_axis',(1.,0.,0.));
#15842=DIRECTION('center_axis',(0.,0.,1.));
#15843=DIRECTION('ref_axis',(1.,0.,0.));
#15844=DIRECTION('center_axis',(0.,0.,1.));
#15845=DIRECTION('ref_axis',(1.,0.,0.));
#15846=DIRECTION('center_axis',(0.,0.,1.));
#15847=DIRECTION('ref_axis',(1.,0.,0.));
#15848=DIRECTION('center_axis',(0.,0.,1.));
#15849=DIRECTION('ref_axis',(1.,0.,0.));
#15850=DIRECTION('center_axis',(0.,0.,1.));
#15851=DIRECTION('ref_axis',(1.,0.,0.));
#15852=DIRECTION('center_axis',(0.,0.,-1.));
#15853=DIRECTION('ref_axis',(1.,0.,0.));
#15854=DIRECTION('center_axis',(0.,0.,-1.));
#15855=DIRECTION('ref_axis',(1.,0.,0.));
#15856=DIRECTION('center_axis',(0.,0.,-1.));
#15857=DIRECTION('ref_axis',(1.,0.,0.));
#15858=DIRECTION('center_axis',(0.,0.,-1.));
#15859=DIRECTION('ref_axis',(1.,0.,0.));
#15860=DIRECTION('center_axis',(0.,0.,1.));
#15861=DIRECTION('ref_axis',(1.,0.,0.));
#15862=DIRECTION('center_axis',(0.,0.,1.));
#15863=DIRECTION('ref_axis',(1.,0.,0.));
#15864=DIRECTION('',(0.,0.,1.));
#15865=DIRECTION('center_axis',(0.,0.,1.));
#15866=DIRECTION('ref_axis',(1.,0.,0.));
#15867=DIRECTION('center_axis',(0.,0.,1.));
#15868=DIRECTION('ref_axis',(1.,0.,0.));
#15869=DIRECTION('',(0.,0.,1.));
#15870=DIRECTION('center_axis',(0.,0.,1.));
#15871=DIRECTION('ref_axis',(1.,0.,0.));
#15872=DIRECTION('center_axis',(0.,0.,1.));
#15873=DIRECTION('ref_axis',(1.,0.,0.));
#15874=DIRECTION('',(0.,0.,1.));
#15875=DIRECTION('center_axis',(0.,0.,1.));
#15876=DIRECTION('ref_axis',(1.,0.,0.));
#15877=DIRECTION('center_axis',(0.,0.,1.));
#15878=DIRECTION('ref_axis',(1.,0.,0.));
#15879=DIRECTION('',(0.,0.,1.));
#15880=DIRECTION('center_axis',(0.,0.,1.));
#15881=DIRECTION('ref_axis',(1.,0.,0.));
#15882=DIRECTION('center_axis',(0.,0.,1.));
#15883=DIRECTION('ref_axis',(1.,0.,0.));
#15884=DIRECTION('',(0.,0.,1.));
#15885=DIRECTION('center_axis',(0.,0.,-1.));
#15886=DIRECTION('ref_axis',(1.,0.,0.));
#15887=DIRECTION('center_axis',(0.,0.,1.));
#15888=DIRECTION('ref_axis',(1.,0.,0.));
#15889=DIRECTION('center_axis',(0.,0.,1.));
#15890=DIRECTION('ref_axis',(1.,0.,0.));
#15891=DIRECTION('center_axis',(0.,0.,1.));
#15892=DIRECTION('ref_axis',(1.,0.,0.));
#15893=DIRECTION('',(0.,0.,-1.));
#15894=DIRECTION('center_axis',(0.,0.,1.));
#15895=DIRECTION('ref_axis',(1.,0.,0.));
#15896=DIRECTION('center_axis',(0.,0.,1.));
#15897=DIRECTION('ref_axis',(1.,0.,0.));
#15898=DIRECTION('',(0.,0.,-1.));
#15899=DIRECTION('center_axis',(0.,0.,-1.));
#15900=DIRECTION('ref_axis',(1.,0.,0.));
#15901=DIRECTION('center_axis',(0.,0.,1.));
#15902=DIRECTION('ref_axis',(1.,0.,0.));
#15903=DIRECTION('center_axis',(0.,0.,1.));
#15904=DIRECTION('ref_axis',(1.,0.,0.));
#19388=CARTESIAN_POINT('',(0.,0.,0.));
#19389=CARTESIAN_POINT('Origin',(1.,0.,5.4));
#19390=CARTESIAN_POINT('',(1.27573508221731,0.25,5.4));
#19391=CARTESIAN_POINT('',(1.3,-3.265531974911E-17,5.65));
#19392=CARTESIAN_POINT('Ctrl Pts',(1.27573508221731,0.25,5.4));
#19393=CARTESIAN_POINT('Ctrl Pts',(1.27573508221731,0.25,5.4314757779847));
#19394=CARTESIAN_POINT('Ctrl Pts',(1.27702069216276,0.243693465283356,5.46499438091527));
#19395=CARTESIAN_POINT('Ctrl Pts',(1.28163032180518,0.218156065105989,5.52656503879345));
#19396=CARTESIAN_POINT('Ctrl Pts',(1.28488408143016,0.198929339789528,5.55462405080375));
#19397=CARTESIAN_POINT('Ctrl Pts',(1.29096514782826,0.15462510881767,5.5989282817756));
#19398=CARTESIAN_POINT('Ctrl Pts',(1.29419244883598,0.126565646309025,5.61815583615436));
#19399=CARTESIAN_POINT('Ctrl Pts',(1.29874124129215,0.0649934270822326,
5.6436938378755));
#19400=CARTESIAN_POINT('Ctrl Pts',(1.3,0.0314742746963997,5.65));
#19401=CARTESIAN_POINT('Ctrl Pts',(1.3,6.24500451351651E-17,5.65));
#19402=CARTESIAN_POINT('Ctrl Pts',(1.3,-3.46944695195361E-17,5.65));
#19403=CARTESIAN_POINT('Ctrl Pts',(1.3,-0.0314742746963997,5.65));
#19404=CARTESIAN_POINT('Ctrl Pts',(1.29874124129215,-0.0649934270822321,
5.6436938378755));
#19405=CARTESIAN_POINT('Ctrl Pts',(1.29419244883598,-0.126565646309024,
5.61815583615436));
#19406=CARTESIAN_POINT('Ctrl Pts',(1.29096514782826,-0.15462510881767,5.5989282817756));
#19407=CARTESIAN_POINT('Ctrl Pts',(1.28488408143016,-0.198929339789528,
5.55462405080375));
#19408=CARTESIAN_POINT('Ctrl Pts',(1.28163032180518,-0.218156065105989,
5.52656503879345));
#19409=CARTESIAN_POINT('Ctrl Pts',(1.27702069216276,-0.243693465283357,
5.46499438091527));
#19410=CARTESIAN_POINT('Ctrl Pts',(1.27573508221731,-0.25,5.4314757779847));
#19411=CARTESIAN_POINT('Ctrl Pts',(1.27573508221731,-0.25,5.3685242220153));
#19412=CARTESIAN_POINT('Ctrl Pts',(1.27702069216276,-0.243693465283357,
5.33500561908473));
#19413=CARTESIAN_POINT('Ctrl Pts',(1.28163032180518,-0.218156065105989,
5.27343496120655));
#19414=CARTESIAN_POINT('Ctrl Pts',(1.28488408143016,-0.198929339789528,
5.24537594919626));
#19415=CARTESIAN_POINT('Ctrl Pts',(1.29096514782826,-0.15462510881767,5.2010717182244));
#19416=CARTESIAN_POINT('Ctrl Pts',(1.29419244883598,-0.126565646309025,
5.18184416384564));
#19417=CARTESIAN_POINT('Ctrl Pts',(1.29874124129215,-0.064993427082233,
5.1563061621245));
#19418=CARTESIAN_POINT('Ctrl Pts',(1.3,-0.0314742746963997,5.15));
#19419=CARTESIAN_POINT('Ctrl Pts',(1.3,0.0314742746963996,5.15));
#19420=CARTESIAN_POINT('Ctrl Pts',(1.29874124129215,0.0649934270822325,
5.1563061621245));
#19421=CARTESIAN_POINT('Ctrl Pts',(1.29419244883598,0.126565646309025,5.18184416384564));
#19422=CARTESIAN_POINT('Ctrl Pts',(1.29096514782826,0.15462510881767,5.2010717182244));
#19423=CARTESIAN_POINT('Ctrl Pts',(1.28488408143016,0.198929339789528,5.24537594919626));
#19424=CARTESIAN_POINT('Ctrl Pts',(1.28163032180518,0.21815606510599,5.27343496120655));
#19425=CARTESIAN_POINT('Ctrl Pts',(1.27702069216276,0.243693465283357,5.33500561908473));
#19426=CARTESIAN_POINT('Ctrl Pts',(1.27573508221731,0.25,5.3685242220153));
#19427=CARTESIAN_POINT('Ctrl Pts',(1.27573508221731,0.25,5.4));
#19428=CARTESIAN_POINT('',(2.2,-3.06161699786838E-17,5.65));
#19429=CARTESIAN_POINT('',(1.,-3.06161699786838E-17,5.65));
#19430=CARTESIAN_POINT('',(2.18574929943944,0.25,5.4));
#19431=CARTESIAN_POINT('Ctrl Pts',(2.18574929943944,0.25,5.4));
#19432=CARTESIAN_POINT('Ctrl Pts',(2.18574929943944,0.25,5.36858020459885));
#19433=CARTESIAN_POINT('Ctrl Pts',(2.1864966418499,0.243715184304782,5.33508482465665));
#19434=CARTESIAN_POINT('Ctrl Pts',(2.18919078893771,0.218193365136867,5.27349811248658));
#19435=CARTESIAN_POINT('Ctrl Pts',(2.19109812170418,0.198957838484313,5.24540444789104));
#19436=CARTESIAN_POINT('Ctrl Pts',(2.19467432003671,0.15459567835042,5.20104228775715));
#19437=CARTESIAN_POINT('Ctrl Pts',(2.19657626523243,0.126501958673344,5.18180666233484));
#19438=CARTESIAN_POINT('Ctrl Pts',(2.19925807248334,0.0649150608388436,
5.15628477026131));
#19439=CARTESIAN_POINT('Ctrl Pts',(2.2,0.0314196165789469,5.15));
#19440=CARTESIAN_POINT('Ctrl Pts',(2.2,-0.0314196165789469,5.15));
#19441=CARTESIAN_POINT('Ctrl Pts',(2.19925807248334,-0.0649150608388436,
5.15628477026131));
#19442=CARTESIAN_POINT('Ctrl Pts',(2.19657626523243,-0.126501958673344,
5.18180666233484));
#19443=CARTESIAN_POINT('Ctrl Pts',(2.19467432003671,-0.15459567835042,5.20104228775715));
#19444=CARTESIAN_POINT('Ctrl Pts',(2.19109812170418,-0.198957838484313,
5.24540444789104));
#19445=CARTESIAN_POINT('Ctrl Pts',(2.18919078893771,-0.218193365136867,
5.27349811248658));
#19446=CARTESIAN_POINT('Ctrl Pts',(2.1864966418499,-0.243715184304782,5.33508482465665));
#19447=CARTESIAN_POINT('Ctrl Pts',(2.18574929943944,-0.25,5.36858020459885));
#19448=CARTESIAN_POINT('Ctrl Pts',(2.18574929943944,-0.25,5.43141979540115));
#19449=CARTESIAN_POINT('Ctrl Pts',(2.1864966418499,-0.243715184304782,5.46491517534335));
#19450=CARTESIAN_POINT('Ctrl Pts',(2.18919078893771,-0.218193365136866,
5.52650188751342));
#19451=CARTESIAN_POINT('Ctrl Pts',(2.19109812170418,-0.198957838484313,
5.55459555210896));
#19452=CARTESIAN_POINT('Ctrl Pts',(2.19467432003671,-0.15459567835042,5.59895771224286));
#19453=CARTESIAN_POINT('Ctrl Pts',(2.19657626523243,-0.126501958673343,
5.61819333766516));
#19454=CARTESIAN_POINT('Ctrl Pts',(2.19925807248334,-0.0649150608388435,
5.64371522973869));
#19455=CARTESIAN_POINT('Ctrl Pts',(2.2,-0.0314196165789469,5.65));
#19456=CARTESIAN_POINT('Ctrl Pts',(2.2,-8.32667268468867E-17,5.65));
#19457=CARTESIAN_POINT('Ctrl Pts',(2.2,6.24500451351651E-17,5.65));
#19458=CARTESIAN_POINT('Ctrl Pts',(2.2,0.0314196165789471,5.65));
#19459=CARTESIAN_POINT('Ctrl Pts',(2.19925807248334,0.0649150608388437,
5.64371522973869));
#19460=CARTESIAN_POINT('Ctrl Pts',(2.19657626523243,0.126501958673344,5.61819333766516));
#19461=CARTESIAN_POINT('Ctrl Pts',(2.19467432003671,0.15459567835042,5.59895771224285));
#19462=CARTESIAN_POINT('Ctrl Pts',(2.19109812170418,0.198957838484313,5.55459555210896));
#19463=CARTESIAN_POINT('Ctrl Pts',(2.18919078893771,0.218193365136867,5.52650188751342));
#19464=CARTESIAN_POINT('Ctrl Pts',(2.1864966418499,0.243715184304782,5.46491517534335));
#19465=CARTESIAN_POINT('Ctrl Pts',(2.18574929943944,0.25,5.43141979540115));
#19466=CARTESIAN_POINT('Ctrl Pts',(2.18574929943944,0.25,5.4));
#19467=CARTESIAN_POINT('Origin',(-1.4142135623731,-1.41421356237309,8.5));
#19468=CARTESIAN_POINT('',(-1.5792135623731,-1.41421356237309,8.5));
#19469=CARTESIAN_POINT('Origin',(-1.4142135623731,-1.41421356237309,8.5));
#19470=CARTESIAN_POINT('',(-1.5792135623731,-1.41421356237309,9.2));
#19471=CARTESIAN_POINT('',(-1.5792135623731,-1.41421356237309,8.5));
#19472=CARTESIAN_POINT('Origin',(-1.4142135623731,-1.41421356237309,9.2));
#19473=CARTESIAN_POINT('Origin',(-1.4142135623731,-1.41421356237309,8.5));
#19474=CARTESIAN_POINT('Origin',(-1.41421356237309,1.4142135623731,8.5));
#19475=CARTESIAN_POINT('',(-1.57921356237309,1.4142135623731,8.5));
#19476=CARTESIAN_POINT('Origin',(-1.41421356237309,1.4142135623731,8.5));
#19477=CARTESIAN_POINT('',(-1.57921356237309,1.4142135623731,9.2));
#19478=CARTESIAN_POINT('',(-1.57921356237309,1.4142135623731,8.5));
#19479=CARTESIAN_POINT('Origin',(-1.41421356237309,1.4142135623731,9.2));
#19480=CARTESIAN_POINT('Origin',(-1.41421356237309,1.4142135623731,8.5));
#19481=CARTESIAN_POINT('Origin',(1.4142135623731,1.41421356237309,8.5));
#19482=CARTESIAN_POINT('',(1.2492135623731,1.41421356237309,8.5));
#19483=CARTESIAN_POINT('Origin',(1.4142135623731,1.41421356237309,8.5));
#19484=CARTESIAN_POINT('',(1.2492135623731,1.41421356237309,9.2));
#19485=CARTESIAN_POINT('',(1.2492135623731,1.41421356237309,8.5));
#19486=CARTESIAN_POINT('Origin',(1.4142135623731,1.41421356237309,9.2));
#19487=CARTESIAN_POINT('Origin',(1.4142135623731,1.41421356237309,8.5));
#19488=CARTESIAN_POINT('Origin',(1.41421356237309,-1.4142135623731,8.5));
#19489=CARTESIAN_POINT('',(1.24921356237309,-1.4142135623731,8.5));
#19490=CARTESIAN_POINT('Origin',(1.41421356237309,-1.4142135623731,8.5));
#19491=CARTESIAN_POINT('',(1.24921356237309,-1.4142135623731,9.2));
#19492=CARTESIAN_POINT('',(1.24921356237309,-1.4142135623731,8.5));
#19493=CARTESIAN_POINT('Origin',(1.41421356237309,-1.4142135623731,9.2));
#19494=CARTESIAN_POINT('Origin',(1.41421356237309,-1.4142135623731,8.5));
#19495=CARTESIAN_POINT('Origin',(-1.76776695296637,-1.76776695296637,1.4));
#19496=CARTESIAN_POINT('',(-1.8139637388702,-1.24480341984751,1.4));
#19497=CARTESIAN_POINT('',(-1.24480341984751,-1.81396373887019,1.4));
#19498=CARTESIAN_POINT('Origin',(0.,0.,1.4));
#19499=CARTESIAN_POINT('Origin',(-1.76776695296637,-1.76776695296637,1.4));
#19500=CARTESIAN_POINT('Origin',(-1.76776695296637,-1.76776695296637,0.8));
#19501=CARTESIAN_POINT('',(-1.8139637388702,-1.24480341984751,0.8));
#19502=CARTESIAN_POINT('',(-1.8139637388702,-1.24480341984751,0.8));
#19503=CARTESIAN_POINT('',(-1.24480341984751,-1.81396373887019,0.8));
#19504=CARTESIAN_POINT('Origin',(-1.76776695296637,-1.76776695296637,0.8));
#19505=CARTESIAN_POINT('',(-1.24480341984751,-1.81396373887019,0.8));
#19506=CARTESIAN_POINT('Origin',(-1.76776695296637,1.76776695296637,0.8));
#19507=CARTESIAN_POINT('',(-1.81396373887019,1.24480341984751,1.4));
#19508=CARTESIAN_POINT('',(-1.81396373887019,1.24480341984751,0.8));
#19509=CARTESIAN_POINT('',(-1.81396373887019,1.24480341984751,0.8));
#19510=CARTESIAN_POINT('',(-1.24480341984751,1.81396373887019,1.4));
#19511=CARTESIAN_POINT('Origin',(-1.76776695296637,1.76776695296637,1.4));
#19512=CARTESIAN_POINT('',(-1.24480341984751,1.81396373887019,0.8));
#19513=CARTESIAN_POINT('',(-1.24480341984751,1.81396373887019,0.8));
#19514=CARTESIAN_POINT('Origin',(-1.76776695296637,1.76776695296637,0.8));
#19515=CARTESIAN_POINT('Origin',(-1.76776695296637,1.76776695296637,1.4));
#19516=CARTESIAN_POINT('Origin',(0.,0.,1.4));
#19517=CARTESIAN_POINT('Origin',(1.76776695296637,1.76776695296637,0.8));
#19518=CARTESIAN_POINT('',(1.24480341984751,1.81396373887019,1.4));
#19519=CARTESIAN_POINT('',(1.24480341984751,1.81396373887019,0.8));
#19520=CARTESIAN_POINT('',(1.24480341984751,1.81396373887019,0.8));
#19521=CARTESIAN_POINT('',(1.81396373887019,1.24480341984751,1.4));
#19522=CARTESIAN_POINT('Origin',(1.76776695296637,1.76776695296637,1.4));
#19523=CARTESIAN_POINT('',(1.81396373887019,1.24480341984751,0.8));
#19524=CARTESIAN_POINT('',(1.81396373887019,1.24480341984751,0.8));
#19525=CARTESIAN_POINT('Origin',(1.76776695296637,1.76776695296637,0.8));
#19526=CARTESIAN_POINT('Origin',(1.76776695296637,1.76776695296637,1.4));
#19527=CARTESIAN_POINT('Origin',(0.,0.,1.4));
#19528=CARTESIAN_POINT('Origin',(1.76776695296637,-1.76776695296637,0.8));
#19529=CARTESIAN_POINT('',(1.81396373887019,-1.24480341984751,1.4));
#19530=CARTESIAN_POINT('',(1.81396373887019,-1.24480341984751,0.8));
#19531=CARTESIAN_POINT('',(1.81396373887019,-1.24480341984751,0.8));
#19532=CARTESIAN_POINT('',(1.24480341984751,-1.8139637388702,1.4));
#19533=CARTESIAN_POINT('Origin',(1.76776695296637,-1.76776695296637,1.4));
#19534=CARTESIAN_POINT('',(1.24480341984751,-1.8139637388702,0.8));
#19535=CARTESIAN_POINT('',(1.24480341984751,-1.8139637388702,0.8));
#19536=CARTESIAN_POINT('Origin',(1.76776695296637,-1.76776695296637,0.8));
#19537=CARTESIAN_POINT('Origin',(1.76776695296637,-1.76776695296637,1.4));
#19538=CARTESIAN_POINT('Origin',(0.,0.,1.4));
#19539=CARTESIAN_POINT('Origin',(0.,0.,0.));
#19540=CARTESIAN_POINT('',(-2.2,-2.69422295812418E-16,9.2));
#19541=CARTESIAN_POINT('Origin',(0.,0.,9.2));
#19542=CARTESIAN_POINT('',(-2.2,-2.69422295812418E-16,0.8));
#19543=CARTESIAN_POINT('',(-2.2,-2.69422295812418E-16,0.));
#19544=CARTESIAN_POINT('Origin',(0.,0.,0.8));
#19545=CARTESIAN_POINT('Origin',(0.,0.,0.8));
#19546=CARTESIAN_POINT('Origin',(0.,0.,0.8));
#19547=CARTESIAN_POINT('Origin',(0.,0.,0.8));
#19548=CARTESIAN_POINT('Origin',(0.,0.,0.8));
#19549=CARTESIAN_POINT('Origin',(0.,0.,0.8));
#19550=CARTESIAN_POINT('',(-3.,-3.67394039744206E-16,0.8));
#19551=CARTESIAN_POINT('Origin',(0.,0.,0.8));
#19552=CARTESIAN_POINT('',(-2.04276695296637,-1.76776695296637,0.8));
#19553=CARTESIAN_POINT('Origin',(-1.76776695296637,-1.76776695296637,0.8));
#19554=CARTESIAN_POINT('',(1.49276695296637,1.76776695296637,0.8));
#19555=CARTESIAN_POINT('Origin',(1.76776695296637,1.76776695296637,0.8));
#19556=CARTESIAN_POINT('',(1.49276695296637,-1.76776695296637,0.8));
#19557=CARTESIAN_POINT('Origin',(1.76776695296637,-1.76776695296637,0.8));
#19558=CARTESIAN_POINT('',(-2.04276695296637,1.76776695296637,0.8));
#19559=CARTESIAN_POINT('Origin',(-1.76776695296637,1.76776695296637,0.8));
#19560=CARTESIAN_POINT('Origin',(-1.76776695296637,-1.76776695296637,-0.1));
#19561=CARTESIAN_POINT('',(-2.04276695296637,-1.76776695296637,0.));
#19562=CARTESIAN_POINT('Origin',(-1.76776695296637,-1.76776695296637,0.));
#19563=CARTESIAN_POINT('',(-2.04276695296637,-1.76776695296637,-0.1));
#19564=CARTESIAN_POINT('Origin',(-1.76776695296637,1.76776695296637,-0.1));
#19565=CARTESIAN_POINT('',(-2.04276695296637,1.76776695296637,0.));
#19566=CARTESIAN_POINT('Origin',(-1.76776695296637,1.76776695296637,0.));
#19567=CARTESIAN_POINT('',(-2.04276695296637,1.76776695296637,-0.1));
#19568=CARTESIAN_POINT('Origin',(1.76776695296637,1.76776695296637,-0.1));
#19569=CARTESIAN_POINT('',(1.49276695296637,1.76776695296637,0.));
#19570=CARTESIAN_POINT('Origin',(1.76776695296637,1.76776695296637,0.));
#19571=CARTESIAN_POINT('',(1.49276695296637,1.76776695296637,-0.1));
#19572=CARTESIAN_POINT('Origin',(1.76776695296637,-1.76776695296637,-0.1));
#19573=CARTESIAN_POINT('',(1.49276695296637,-1.76776695296637,0.));
#19574=CARTESIAN_POINT('Origin',(1.76776695296637,-1.76776695296637,0.));
#19575=CARTESIAN_POINT('',(1.49276695296637,-1.76776695296637,-0.1));
#19576=CARTESIAN_POINT('Origin',(0.,0.,6.));
#19577=CARTESIAN_POINT('',(-1.6,-1.95943487863577E-16,6.));
#19578=CARTESIAN_POINT('Origin',(0.,0.,6.));
#19579=CARTESIAN_POINT('',(-1.6,1.95943487863577E-16,9.2));
#19580=CARTESIAN_POINT('',(-1.6,-1.95943487863577E-16,6.));
#19581=CARTESIAN_POINT('Origin',(0.,0.,9.2));
#19582=CARTESIAN_POINT('Origin',(0.,0.,6.));
#19583=CARTESIAN_POINT('',(-1.3,-1.59204083889156E-16,6.));
#19584=CARTESIAN_POINT('Origin',(0.,0.,6.));
#19585=CARTESIAN_POINT('Origin',(0.,0.,0.));
#19586=CARTESIAN_POINT('',(-3.,-3.67394039744206E-16,0.));
#19587=CARTESIAN_POINT('',(-3.,-3.67394039744206E-16,0.));
#19588=CARTESIAN_POINT('Origin',(0.,0.,0.));
#19589=CARTESIAN_POINT('Origin',(0.,0.,0.));
#19590=CARTESIAN_POINT('',(-1.3,-1.59204083889156E-16,0.));
#19591=CARTESIAN_POINT('',(-1.3,-1.59204083889156E-16,0.));
#19592=CARTESIAN_POINT('Origin',(0.,0.,0.));
#19593=CARTESIAN_POINT('Origin',(0.,0.,9.2));
#19594=CARTESIAN_POINT('Origin',(0.,0.,0.));
#57788=UNCERTAINTY_MEASURE_WITH_UNIT(LENGTH_MEASURE(0.001),#57901,
'DISTANCE_ACCURACY_VALUE',
'Maximum model space distance between geometric entities at asserted c
onnectivities');
#57841=UNCERTAINTY_MEASURE_WITH_UNIT(LENGTH_MEASURE(0.001),#57901,
'DISTANCE_ACCURACY_VALUE',
'Maximum model space distance between geometric entities at asserted c
onnectivities');
#57847=(
GEOMETRIC_REPRESENTATION_CONTEXT(3)
GLOBAL_UNCERTAINTY_ASSIGNED_CONTEXT((#57788))
GLOBAL_UNIT_ASSIGNED_CONTEXT((#57901,#57903,#57904))
REPRESENTATION_CONTEXT('','3D')
);
#57900=(
GEOMETRIC_REPRESENTATION_CONTEXT(3)
GLOBAL_UNCERTAINTY_ASSIGNED_CONTEXT((#57841))
GLOBAL_UNIT_ASSIGNED_CONTEXT((#57901,#57903,#57904))
REPRESENTATION_CONTEXT('','3D')
);
#57901=(
LENGTH_UNIT()
NAMED_UNIT(*)
SI_UNIT(.CENTI.,.METRE.)
);
#57903=(
NAMED_UNIT(*)
PLANE_ANGLE_UNIT()
SI_UNIT($,.RADIAN.)
);
#57904=(
NAMED_UNIT(*)
SI_UNIT($,.STERADIAN.)
SOLID_ANGLE_UNIT()
);
#57910=SHAPE_DEFINITION_REPRESENTATION(#57968,#58114);
#57968=PRODUCT_DEFINITION_SHAPE('',$,#58173);
#58114=SHAPE_REPRESENTATION('',(#14254),#57847);
#58167=PRODUCT_DEFINITION_CONTEXT('part definition',#58343,'design');
#58173=PRODUCT_DEFINITION('Input bearing post','Input bearing post',#58231,
#58167);
#58231=PRODUCT_DEFINITION_FORMATION('',$,#58350);
#58343=APPLICATION_CONTEXT(
'Core Data for Automotive Mechanical Design Process');
#58344=PRODUCT_CONTEXT('part definition',#58343,'mechanical');
#58350=PRODUCT('Input bearing post','Input bearing post',
'Input bearing post',(#58344));
#58459=COLOUR_RGB('Grey',0.48,0.52,0.57);
#58460=FILL_AREA_STYLE_COLOUR('',#58459);
#58461=FILL_AREA_STYLE('',(#58460));
#58462=SURFACE_STYLE_FILL_AREA(#58461);
#58463=SURFACE_SIDE_STYLE('',(#58462));
#58464=SURFACE_STYLE_USAGE(.BOTH.,#58463);
#58465=PRESENTATION_STYLE_ASSIGNMENT((#58464));
ENDSEC;
END-ISO-10303-21;
